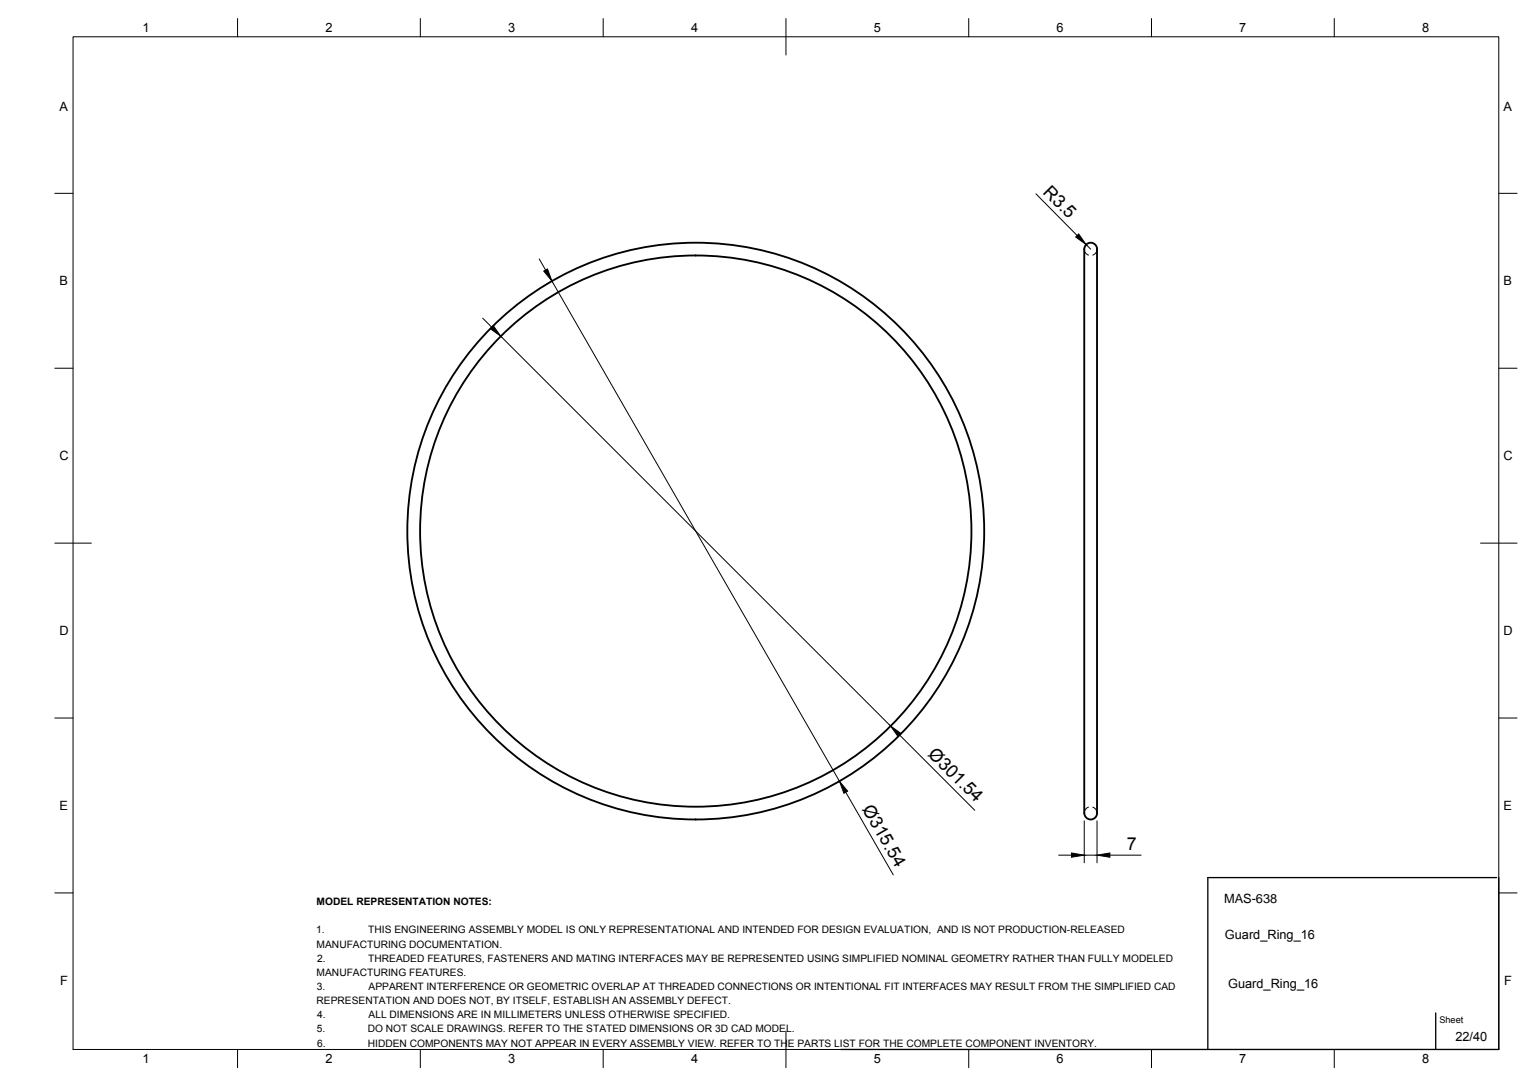
ISO-10303-21;
HEADER;
FILE_DESCRIPTION((''),'2;1');
FILE_NAME('Guard_Ring_16.step','2026-10-09T12:00:21-07:00',(''),(''),'','','');
FILE_SCHEMA (('AUTOMOTIVE_DESIGN { 1 0 10303 214 3 1 1 }'));
ENDSEC;
DATA;
#10=MECHANICAL_DESIGN_GEOMETRIC_PRESENTATION_REPRESENTATION('',(#420,#421),#10334);
#349=SHAPE_REPRESENTATION_RELATIONSHIP('SRR','None',#10465,#381) ;
#381=ADVANCED_BREP_SHAPE_REPRESENTATION('',(#453),#10317) ;
#420=STYLED_ITEM('',(#10631),#3382) ;
#421=STYLED_ITEM('',(#10632),#453) ;
#453=MANIFOLD_SOLID_BREP('Body1',#3575) ;
#874=FACE_OUTER_BOUND('',#1074,.T.) ;
#1074=EDGE_LOOP('',(#2409,#2410,#2411,#2412)) ;
#1306=CIRCLE('',#4035,0.349999999999999) ;
#1307=CIRCLE('',#4036,15.0768144613668) ;
#1528=VERTEX_POINT('',#5728) ;
#1861=EDGE_CURVE('',#1528,#1528,#1306,.T.) ;
#1862=EDGE_CURVE('',#1528,#1528,#1307,.T.) ;
#2409=ORIENTED_EDGE('',*,*,#1861,.F.) ;
#2410=ORIENTED_EDGE('',*,*,#1862,.T.) ;
#2411=ORIENTED_EDGE('',*,*,#1861,.T.) ;
#2412=ORIENTED_EDGE('',*,*,#1862,.F.) ;
#3320=TOROIDAL_SURFACE('',#4034,15.4268144613668,0.349999999999999) ;
#3382=ADVANCED_FACE('',(#874),#3320,.T.) ;
#3575=CLOSED_SHELL('',(#3382)) ;
#4033=AXIS2_PLACEMENT_3D('',#5726,#4627,#4628) ;
#4034=AXIS2_PLACEMENT_3D('',#5727,#4629,#4630) ;
#4035=AXIS2_PLACEMENT_3D('',#5729,#4631,#4632) ;
#4036=AXIS2_PLACEMENT_3D('',#5730,#4633,#4634) ;
#4627=DIRECTION('axis',(0.,0.,1.)) ;
#4628=DIRECTION('refdir',(1.,0.,0.)) ;
#4629=DIRECTION('center_axis',(-6.42891162084177E-17,-1.,-1.01883556321148E-16)) ;
#4630=DIRECTION('ref_axis',(1.,0.,0.)) ;
#4631=DIRECTION('center_axis',(0.,1.01883556321148E-16,-1.)) ;
#4632=DIRECTION('ref_axis',(-1.,0.,0.)) ;
#4633=DIRECTION('center_axis',(6.42891162084177E-17,1.,1.01883556321148E-16)) ;
#4634=DIRECTION('ref_axis',(1.,-6.42891162084177E-17,-6.55000379205715E-33)) ;
#5726=CARTESIAN_POINT('',(0.,0.,0.)) ;
#5727=CARTESIAN_POINT('Origin',(23.47768801576,66.6831179463143,68.2224337400009)) ;
#5728=CARTESIAN_POINT('',(8.4008735543932,66.6831179463143,68.2224337400009)) ;
#5729=CARTESIAN_POINT('Origin',(8.0508735543932,66.6831179463143,68.2224337400009)) ;
#5730=CARTESIAN_POINT('Origin',(23.47768801576,66.6831179463143,68.2224337400009)) ;
#10280=UNCERTAINTY_MEASURE_WITH_UNIT(LENGTH_MEASURE(0.001),#10335,
'DISTANCE_ACCURACY_VALUE',
'Maximum model space distance between geometric entities at asserted c
onnectivities') ;
#10297=UNCERTAINTY_MEASURE_WITH_UNIT(LENGTH_MEASURE(0.001),#10335,
'DISTANCE_ACCURACY_VALUE',
'Maximum model space distance between geometric entities at asserted c
onnectivities') ;
#10317=(
GEOMETRIC_REPRESENTATION_CONTEXT(3)
GLOBAL_UNCERTAINTY_ASSIGNED_CONTEXT((#10280))
GLOBAL_UNIT_ASSIGNED_CONTEXT((#10335,#10337,#10338))
REPRESENTATION_CONTEXT('','3D')
) ;
#10334=(
GEOMETRIC_REPRESENTATION_CONTEXT(3)
GLOBAL_UNCERTAINTY_ASSIGNED_CONTEXT((#10297))
GLOBAL_UNIT_ASSIGNED_CONTEXT((#10335,#10337,#10338))
REPRESENTATION_CONTEXT('','3D')
) ;
#10335=(
LENGTH_UNIT()
NAMED_UNIT(*)
SI_UNIT(.CENTI.,.METRE.)
) ;
#10337=(
NAMED_UNIT(*)
PLANE_ANGLE_UNIT()
SI_UNIT($,.RADIAN.)
) ;
#10338=(
NAMED_UNIT(*)
SI_UNIT($,.STERADIAN.)
SOLID_ANGLE_UNIT()
) ;
#10358=SHAPE_DEFINITION_REPRESENTATION(#10394,#10465) ;
#10394=PRODUCT_DEFINITION_SHAPE('',$,#10502) ;
#10465=SHAPE_REPRESENTATION('',(#4033),#10317) ;
#10482=PRODUCT_DEFINITION_CONTEXT('part definition',#10592,'design') ;
#10502=PRODUCT_DEFINITION('Guard_Ring_16','Guard_Ring_16',#10538,#10482) ;
#10538=PRODUCT_DEFINITION_FORMATION('',$,#10613) ;
#10592=APPLICATION_CONTEXT(
'Core Data for Automotive Mechanical Design Process') ;
#10593=PRODUCT_CONTEXT('part definition',#10592,'mechanical') ;
#10613=PRODUCT('Guard_Ring_16','Guard_Ring_16',$,(#10593)) ;
#10631=PRESENTATION_STYLE_ASSIGNMENT((#10635)) ;
#10632=PRESENTATION_STYLE_ASSIGNMENT((#10636)) ;
#10635=SURFACE_STYLE_USAGE(.BOTH.,#10639) ;
#10636=SURFACE_STYLE_USAGE(.BOTH.,#10640) ;
#10639=SURFACE_SIDE_STYLE('',(#10643)) ;
#10640=SURFACE_SIDE_STYLE('',(#10644)) ;
#10643=SURFACE_STYLE_FILL_AREA(#10647) ;
#10644=SURFACE_STYLE_FILL_AREA(#10648) ;
#10647=FILL_AREA_STYLE('Opaque(25,25,25)',(#10651)) ;
#10648=FILL_AREA_STYLE('Opaque(202,209,238)',(#10652)) ;
#10651=FILL_AREA_STYLE_COLOUR('Opaque(25,25,25)',#10655) ;
#10652=FILL_AREA_STYLE_COLOUR('Opaque(202,209,238)',#10656) ;
#10655=COLOUR_RGB('Opaque(25,25,25)', 0.09019608, 0.27058824, 0.51372549) ;
#10656=COLOUR_RGB('Opaque(202,209,238)', 0.40784314, 0.44705882, 0.49803922) ;
ENDSEC;
END-ISO-10303-21;
